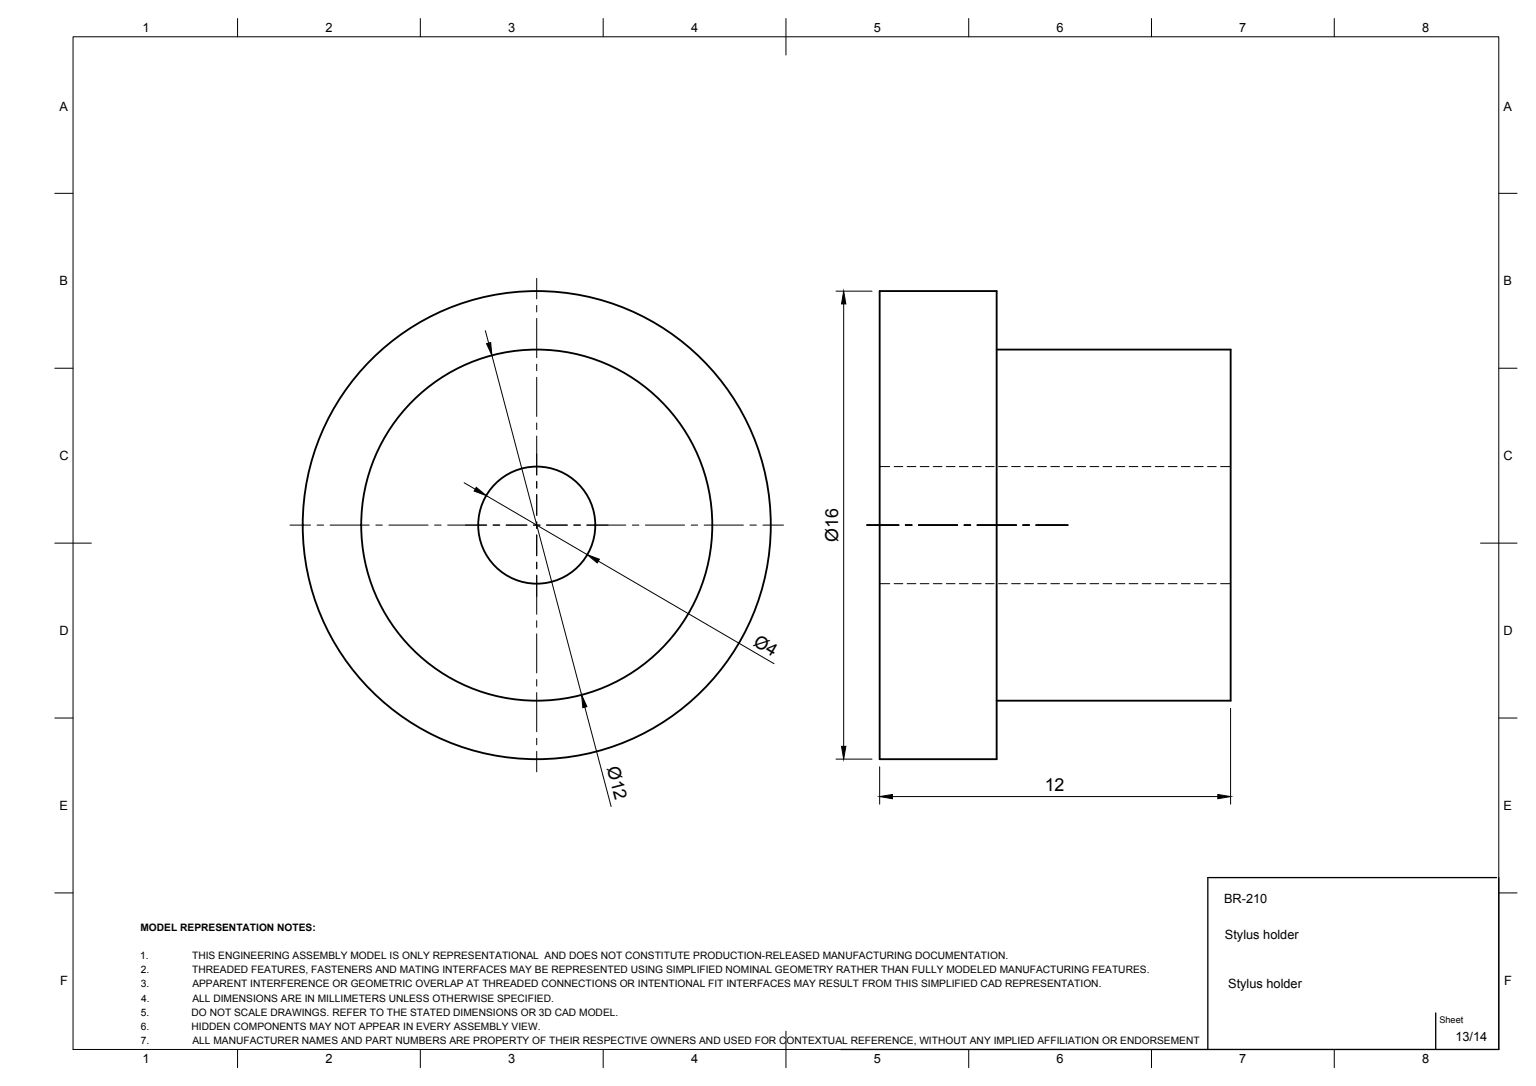
ISO-10303-21;
HEADER;
/* Generated by software containing ST-Developer
 * from STEP Tools, Inc. (www.steptools.com) 
 */

FILE_DESCRIPTION(
/* description */ ('Independent 1:2 reduction pantograph. 120 mm parallelogram sides; fix
ed fulcrum on the extension of a 240 mm link. Drawing point halfway al
ong its link, so its XY displacement is one half of the tracing point.
 Replaceable pivot bushes and retained pins. Calibration and productio
n accuracy unassigned.'),
/* implementation_level */ '2;1');

FILE_NAME(
/* name */ 'Stylus holder.step',
/* time_stamp */ '2026-11-07T22:11:57-08:00',
/* author */ (''),
/* organization */ (''),
/* preprocessor_version */ 'ST-DEVELOPER v20.2',
/* originating_system */ 'Autodesk Translation Framework v15.17.0.0',
/* authorisation */ '');

FILE_SCHEMA (('AUTOMOTIVE_DESIGN { 1 0 10303 214 3 1 1 }'));
ENDSEC;

DATA;
#10=MECHANICAL_DESIGN_GEOMETRIC_PRESENTATION_REPRESENTATION('',(#192),#2926);
#166=SHAPE_REPRESENTATION_RELATIONSHIP('SRR','None',#3003,#179);
#179=ADVANCED_BREP_SHAPE_REPRESENTATION('',(#205),#2919);
#192=STYLED_ITEM('',(#3076),#205);
#205=MANIFOLD_SOLID_BREP('Body1',#1547);
#244=FACE_BOUND('',#482,.T.);
#245=FACE_BOUND('',#485,.T.);
#246=FACE_BOUND('',#489,.T.);
#284=PLANE('',#1810);
#285=PLANE('',#1815);
#286=PLANE('',#1821);
#357=FACE_OUTER_BOUND('',#481,.T.);
#358=FACE_OUTER_BOUND('',#483,.T.);
#359=FACE_OUTER_BOUND('',#484,.T.);
#360=FACE_OUTER_BOUND('',#486,.T.);
#361=FACE_OUTER_BOUND('',#487,.T.);
#362=FACE_OUTER_BOUND('',#488,.T.);
#481=EDGE_LOOP('',(#1271));
#482=EDGE_LOOP('',(#1272));
#483=EDGE_LOOP('',(#1273,#1274,#1275,#1276));
#484=EDGE_LOOP('',(#1277));
#485=EDGE_LOOP('',(#1278));
#486=EDGE_LOOP('',(#1279,#1280,#1281,#1282));
#487=EDGE_LOOP('',(#1283,#1284,#1285,#1286));
#488=EDGE_LOOP('',(#1287));
#489=EDGE_LOOP('',(#1288));
#585=LINE('',#2710,#666);
#586=LINE('',#2716,#667);
#587=LINE('',#2720,#668);
#666=VECTOR('',#2213,8.);
#667=VECTOR('',#2220,2.);
#668=VECTOR('',#2225,6.);
#749=CIRCLE('',#1811,8.);
#750=CIRCLE('',#1812,6.);
#751=CIRCLE('',#1814,8.);
#752=CIRCLE('',#1816,2.);
#753=CIRCLE('',#1818,2.);
#754=CIRCLE('',#1820,6.);
#853=VERTEX_POINT('',#2703);
#854=VERTEX_POINT('',#2705);
#855=VERTEX_POINT('',#2708);
#856=VERTEX_POINT('',#2712);
#857=VERTEX_POINT('',#2715);
#858=VERTEX_POINT('',#2719);
#1000=EDGE_CURVE('',#853,#853,#749,.T.);
#1001=EDGE_CURVE('',#854,#854,#750,.T.);
#1002=EDGE_CURVE('',#855,#855,#751,.T.);
#1003=EDGE_CURVE('',#855,#853,#585,.T.);
#1004=EDGE_CURVE('',#856,#856,#752,.T.);
#1005=EDGE_CURVE('',#856,#857,#586,.T.);
#1006=EDGE_CURVE('',#857,#857,#753,.T.);
#1007=EDGE_CURVE('',#854,#858,#587,.T.);
#1008=EDGE_CURVE('',#858,#858,#754,.T.);
#1271=ORIENTED_EDGE('',*,*,#1000,.F.);
#1272=ORIENTED_EDGE('',*,*,#1001,.T.);
#1273=ORIENTED_EDGE('',*,*,#1002,.F.);
#1274=ORIENTED_EDGE('',*,*,#1003,.T.);
#1275=ORIENTED_EDGE('',*,*,#1000,.T.);
#1276=ORIENTED_EDGE('',*,*,#1003,.F.);
#1277=ORIENTED_EDGE('',*,*,#1002,.T.);
#1278=ORIENTED_EDGE('',*,*,#1004,.T.);
#1279=ORIENTED_EDGE('',*,*,#1004,.F.);
#1280=ORIENTED_EDGE('',*,*,#1005,.T.);
#1281=ORIENTED_EDGE('',*,*,#1006,.T.);
#1282=ORIENTED_EDGE('',*,*,#1005,.F.);
#1283=ORIENTED_EDGE('',*,*,#1001,.F.);
#1284=ORIENTED_EDGE('',*,*,#1007,.T.);
#1285=ORIENTED_EDGE('',*,*,#1008,.T.);
#1286=ORIENTED_EDGE('',*,*,#1007,.F.);
#1287=ORIENTED_EDGE('',*,*,#1008,.F.);
#1288=ORIENTED_EDGE('',*,*,#1006,.F.);
#1431=CYLINDRICAL_SURFACE('',#1813,8.);
#1432=CYLINDRICAL_SURFACE('',#1817,2.);
#1433=CYLINDRICAL_SURFACE('',#1819,6.);
#1501=ADVANCED_FACE('',(#357,#244),#284,.F.);
#1502=ADVANCED_FACE('',(#358),#1431,.T.);
#1503=ADVANCED_FACE('',(#359,#245),#285,.T.);
#1504=ADVANCED_FACE('',(#360),#1432,.F.);
#1505=ADVANCED_FACE('',(#361),#1433,.T.);
#1506=ADVANCED_FACE('',(#362,#246),#286,.F.);
#1547=CLOSED_SHELL('',(#1501,#1502,#1503,#1504,#1505,#1506));
#1809=AXIS2_PLACEMENT_3D('',#2701,#2201,#2202);
#1810=AXIS2_PLACEMENT_3D('',#2702,#2203,#2204);
#1811=AXIS2_PLACEMENT_3D('',#2704,#2205,#2206);
#1812=AXIS2_PLACEMENT_3D('',#2706,#2207,#2208);
#1813=AXIS2_PLACEMENT_3D('',#2707,#2209,#2210);
#1814=AXIS2_PLACEMENT_3D('',#2709,#2211,#2212);
#1815=AXIS2_PLACEMENT_3D('',#2711,#2214,#2215);
#1816=AXIS2_PLACEMENT_3D('',#2713,#2216,#2217);
#1817=AXIS2_PLACEMENT_3D('',#2714,#2218,#2219);
#1818=AXIS2_PLACEMENT_3D('',#2717,#2221,#2222);
#1819=AXIS2_PLACEMENT_3D('',#2718,#2223,#2224);
#1820=AXIS2_PLACEMENT_3D('',#2721,#2226,#2227);
#1821=AXIS2_PLACEMENT_3D('',#2722,#2228,#2229);
#2201=DIRECTION('axis',(0.,0.,1.));
#2202=DIRECTION('refdir',(1.,0.,0.));
#2203=DIRECTION('center_axis',(0.,0.,1.));
#2204=DIRECTION('ref_axis',(1.,0.,0.));
#2205=DIRECTION('center_axis',(0.,0.,1.));
#2206=DIRECTION('ref_axis',(1.,0.,0.));
#2207=DIRECTION('center_axis',(0.,0.,1.));
#2208=DIRECTION('ref_axis',(1.,0.,0.));
#2209=DIRECTION('center_axis',(0.,0.,1.));
#2210=DIRECTION('ref_axis',(1.,0.,0.));
#2211=DIRECTION('center_axis',(0.,0.,1.));
#2212=DIRECTION('ref_axis',(1.,0.,0.));
#2213=DIRECTION('',(0.,0.,-1.));
#2214=DIRECTION('center_axis',(0.,0.,1.));
#2215=DIRECTION('ref_axis',(1.,0.,0.));
#2216=DIRECTION('center_axis',(0.,0.,-1.));
#2217=DIRECTION('ref_axis',(1.,0.,0.));
#2218=DIRECTION('center_axis',(0.,0.,1.));
#2219=DIRECTION('ref_axis',(1.,0.,0.));
#2220=DIRECTION('',(0.,0.,-1.));
#2221=DIRECTION('center_axis',(0.,0.,-1.));
#2222=DIRECTION('ref_axis',(1.,0.,0.));
#2223=DIRECTION('center_axis',(0.,0.,1.));
#2224=DIRECTION('ref_axis',(1.,0.,0.));
#2225=DIRECTION('',(0.,0.,-1.));
#2226=DIRECTION('center_axis',(0.,0.,1.));
#2227=DIRECTION('ref_axis',(1.,0.,0.));
#2228=DIRECTION('center_axis',(0.,0.,1.));
#2229=DIRECTION('ref_axis',(1.,0.,0.));
#2701=CARTESIAN_POINT('',(0.,0.,0.));
#2702=CARTESIAN_POINT('Origin',(0.,0.,8.));
#2703=CARTESIAN_POINT('',(-8.,-9.79717439317883E-16,8.));
#2704=CARTESIAN_POINT('Origin',(0.,0.,8.));
#2705=CARTESIAN_POINT('',(-6.,-7.34788079488412E-16,8.));
#2706=CARTESIAN_POINT('Origin',(0.,0.,8.));
#2707=CARTESIAN_POINT('Origin',(0.,0.,8.));
#2708=CARTESIAN_POINT('',(-8.,-9.79717439317883E-16,12.));
#2709=CARTESIAN_POINT('Origin',(0.,0.,12.));
#2710=CARTESIAN_POINT('',(-8.,-9.79717439317883E-16,8.));
#2711=CARTESIAN_POINT('Origin',(0.,0.,12.));
#2712=CARTESIAN_POINT('',(-2.,-2.44929359829471E-16,12.));
#2713=CARTESIAN_POINT('Origin',(0.,0.,12.));
#2714=CARTESIAN_POINT('Origin',(0.,0.,0.));
#2715=CARTESIAN_POINT('',(-2.,-2.44929359829471E-16,0.));
#2716=CARTESIAN_POINT('',(-2.,-2.44929359829471E-16,0.));
#2717=CARTESIAN_POINT('Origin',(0.,0.,0.));
#2718=CARTESIAN_POINT('Origin',(0.,0.,0.));
#2719=CARTESIAN_POINT('',(-6.,-7.34788079488412E-16,0.));
#2720=CARTESIAN_POINT('',(-6.,-7.34788079488412E-16,0.));
#2721=CARTESIAN_POINT('Origin',(0.,0.,0.));
#2722=CARTESIAN_POINT('Origin',(0.,0.,0.));
#2904=UNCERTAINTY_MEASURE_WITH_UNIT(LENGTH_MEASURE(0.01),#2927,
'DISTANCE_ACCURACY_VALUE',
'Maximum model space distance between geometric entities at asserted c
onnectivities');
#2911=UNCERTAINTY_MEASURE_WITH_UNIT(LENGTH_MEASURE(0.01),#2927,
'DISTANCE_ACCURACY_VALUE',
'Maximum model space distance between geometric entities at asserted c
onnectivities');
#2919=(
GEOMETRIC_REPRESENTATION_CONTEXT(3)
GLOBAL_UNCERTAINTY_ASSIGNED_CONTEXT((#2904))
GLOBAL_UNIT_ASSIGNED_CONTEXT((#2927,#2929,#2930))
REPRESENTATION_CONTEXT('','3D')
);
#2926=(
GEOMETRIC_REPRESENTATION_CONTEXT(3)
GLOBAL_UNCERTAINTY_ASSIGNED_CONTEXT((#2911))
GLOBAL_UNIT_ASSIGNED_CONTEXT((#2927,#2929,#2930))
REPRESENTATION_CONTEXT('','3D')
);
#2927=(
LENGTH_UNIT()
NAMED_UNIT(*)
SI_UNIT(.MILLI.,.METRE.)
);
#2929=(
NAMED_UNIT(*)
PLANE_ANGLE_UNIT()
SI_UNIT($,.RADIAN.)
);
#2930=(
NAMED_UNIT(*)
SI_UNIT($,.STERADIAN.)
SOLID_ANGLE_UNIT()
);
#2938=SHAPE_DEFINITION_REPRESENTATION(#2952,#3003);
#2952=PRODUCT_DEFINITION_SHAPE('',$,#3018);
#3003=SHAPE_REPRESENTATION('',(#1809),#2919);
#3010=PRODUCT_DEFINITION_CONTEXT('part definition',#3054,'design');
#3018=PRODUCT_DEFINITION('Stylus holder','Stylus holder',#3032,#3010);
#3032=PRODUCT_DEFINITION_FORMATION('',$,#3063);
#3054=APPLICATION_CONTEXT(
'Core Data for Automotive Mechanical Design Process');
#3055=PRODUCT_CONTEXT('part definition',#3054,'mechanical');
#3063=PRODUCT('Stylus holder','Stylus holder',$,(#3055));
#3076=PRESENTATION_STYLE_ASSIGNMENT((#3088));
#3088=SURFACE_STYLE_USAGE(.BOTH.,#3100);
#3100=SURFACE_SIDE_STYLE('',(#3112));
#3112=SURFACE_STYLE_FILL_AREA(#3124);
#3124=FILL_AREA_STYLE('Holder gray',(#3136));
#3136=FILL_AREA_STYLE_COLOUR('Holder gray',#3148);
#3148=COLOUR_RGB('Holder gray',0.407843137254902,0.447058823529412,0.498039215686275);
ENDSEC;
END-ISO-10303-21;
